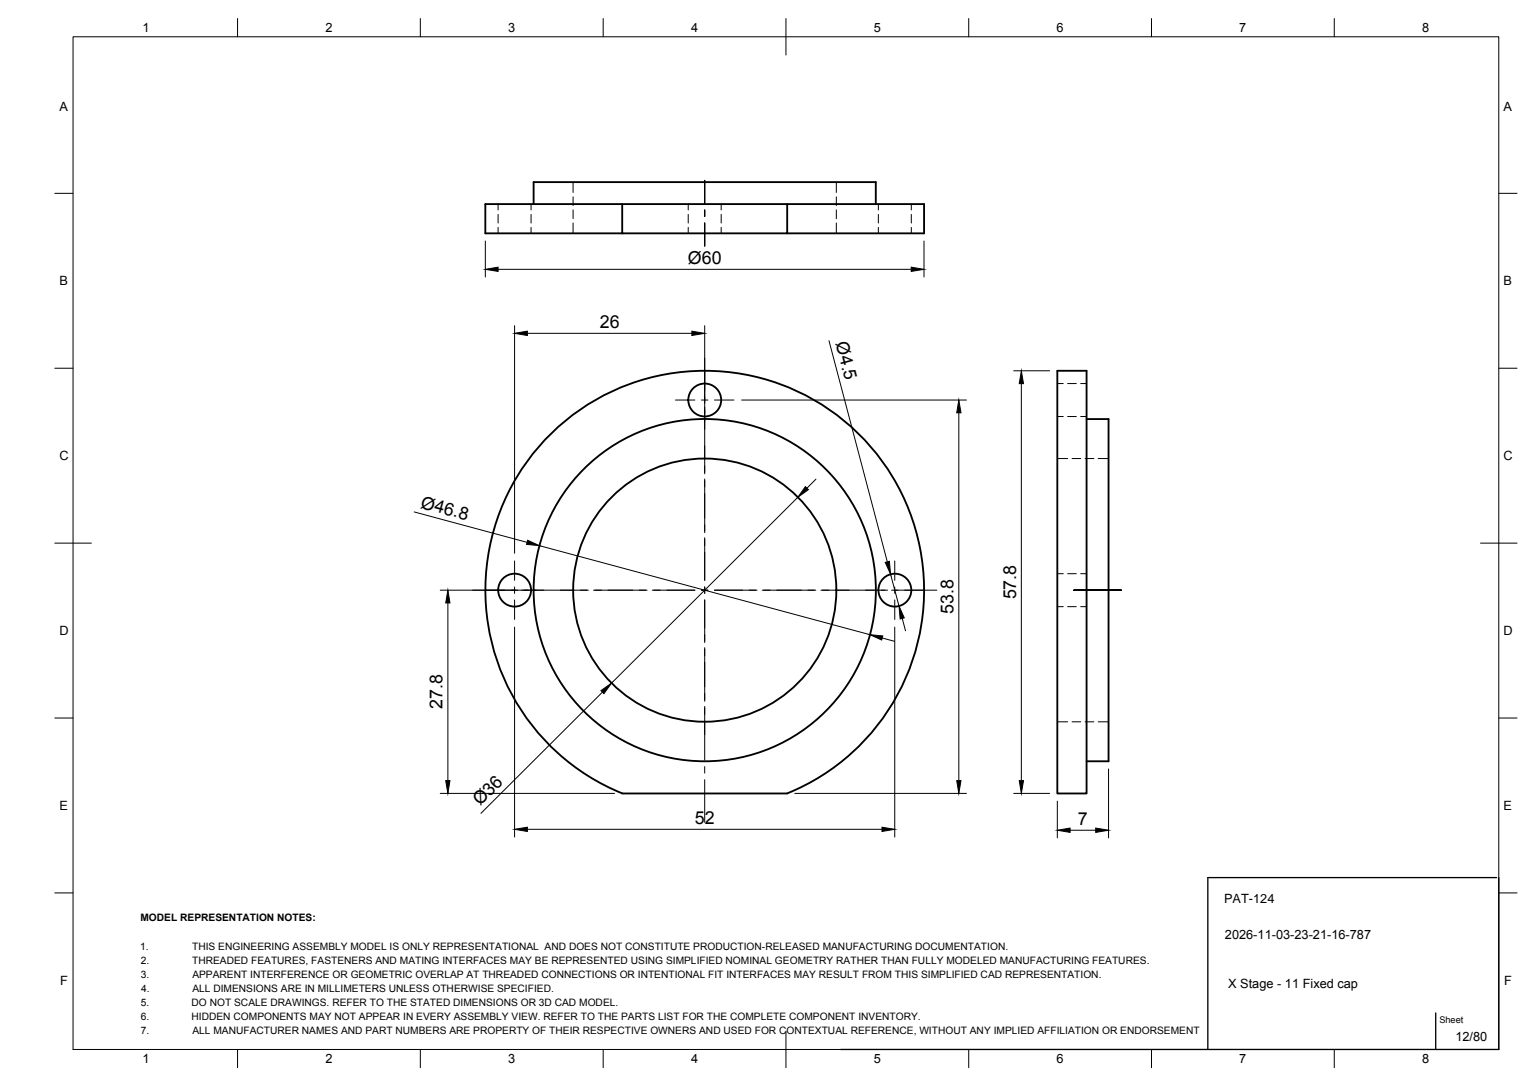
ISO-10303-21;
HEADER;
/* Generated by software containing ST-Developer
 * from STEP Tools, Inc. (www.steptools.com) 
 */

FILE_DESCRIPTION(
/* description */ ('XY cross-slide table'),
/* implementation_level */ '2;1');

FILE_NAME(
/* name */ 'X Stage - 11 Fixed cap.step',
/* time_stamp */ '2026-10-28T03:22:46-07:00',
/* author */ (''),
/* organization */ (''),
/* preprocessor_version */ 'ST-DEVELOPER v20.2',
/* originating_system */ 'Autodesk Translation Framework v15.17.0.0',
/* authorisation */ '');

FILE_SCHEMA (('AUTOMOTIVE_DESIGN { 1 0 10303 214 3 1 1 }'));
ENDSEC;

DATA;
#10=MECHANICAL_DESIGN_GEOMETRIC_PRESENTATION_REPRESENTATION('',(#1677),#62984);
#1511=SHAPE_REPRESENTATION_RELATIONSHIP('SRR','None',#63359,#1594);
#1594=ADVANCED_BREP_SHAPE_REPRESENTATION('',(#1790),#62896);
#1677=STYLED_ITEM('',(#63926),#1790);
#1790=MANIFOLD_SOLID_BREP('Body1',#22971);
#1956=FACE_BOUND('',#4350,.T.);
#1957=FACE_BOUND('',#4351,.T.);
#1958=FACE_BOUND('',#4352,.T.);
#1959=FACE_BOUND('',#4353,.T.);
#1960=FACE_BOUND('',#4357,.T.);
#1961=FACE_BOUND('',#4360,.T.);
#1962=FACE_BOUND('',#4361,.T.);
#1963=FACE_BOUND('',#4362,.T.);
#1964=FACE_BOUND('',#4363,.T.);
#2345=PLANE('',#24201);
#2346=PLANE('',#24202);
#2347=PLANE('',#24209);
#2348=PLANE('',#24213);
#2962=FACE_OUTER_BOUND('',#4345,.T.);
#2963=FACE_OUTER_BOUND('',#4346,.T.);
#2964=FACE_OUTER_BOUND('',#4347,.T.);
#2965=FACE_OUTER_BOUND('',#4348,.T.);
#2966=FACE_OUTER_BOUND('',#4349,.T.);
#2967=FACE_OUTER_BOUND('',#4354,.T.);
#2968=FACE_OUTER_BOUND('',#4355,.T.);
#2969=FACE_OUTER_BOUND('',#4356,.T.);
#2970=FACE_OUTER_BOUND('',#4358,.T.);
#2971=FACE_OUTER_BOUND('',#4359,.T.);
#4345=EDGE_LOOP('',(#15320,#15321,#15322,#15323));
#4346=EDGE_LOOP('',(#15324,#15325,#15326,#15327));
#4347=EDGE_LOOP('',(#15328,#15329,#15330,#15331));
#4348=EDGE_LOOP('',(#15332,#15333,#15334,#15335));
#4349=EDGE_LOOP('',(#15336,#15337));
#4350=EDGE_LOOP('',(#15338));
#4351=EDGE_LOOP('',(#15339));
#4352=EDGE_LOOP('',(#15340));
#4353=EDGE_LOOP('',(#15341));
#4354=EDGE_LOOP('',(#15342,#15343,#15344,#15345));
#4355=EDGE_LOOP('',(#15346,#15347,#15348,#15349));
#4356=EDGE_LOOP('',(#15350));
#4357=EDGE_LOOP('',(#15351));
#4358=EDGE_LOOP('',(#15352,#15353,#15354,#15355));
#4359=EDGE_LOOP('',(#15356,#15357));
#4360=EDGE_LOOP('',(#15358));
#4361=EDGE_LOOP('',(#15359));
#4362=EDGE_LOOP('',(#15360));
#4363=EDGE_LOOP('',(#15361));
#6026=LINE('',#33322,#7513);
#6027=LINE('',#33328,#7514);
#6028=LINE('',#33334,#7515);
#6029=LINE('',#33339,#7516);
#6030=LINE('',#33341,#7517);
#6031=LINE('',#33343,#7518);
#6032=LINE('',#33344,#7519);
#6033=LINE('',#33353,#7520);
#6034=LINE('',#33361,#7521);
#7513=VECTOR('',#26969,0.225);
#7514=VECTOR('',#26976,0.225);
#7515=VECTOR('',#26983,0.225);
#7516=VECTOR('',#26988,1.);
#7517=VECTOR('',#26989,1.);
#7518=VECTOR('',#26990,1.);
#7519=VECTOR('',#26991,1.);
#7520=VECTOR('',#27004,2.34);
#7521=VECTOR('',#27015,1.8);
#8968=CIRCLE('',#24193,0.225);
#8969=CIRCLE('',#24194,0.225);
#8970=CIRCLE('',#24196,0.225);
#8971=CIRCLE('',#24197,0.225);
#8972=CIRCLE('',#24199,0.225);
#8973=CIRCLE('',#24200,0.225);
#8974=CIRCLE('',#24203,3.);
#8975=CIRCLE('',#24204,2.34);
#8976=CIRCLE('',#24206,3.);
#8977=CIRCLE('',#24208,2.34);
#8978=CIRCLE('',#24210,1.8);
#8979=CIRCLE('',#24212,1.8);
#9909=VERTEX_POINT('',#33319);
#9910=VERTEX_POINT('',#33321);
#9911=VERTEX_POINT('',#33325);
#9912=VERTEX_POINT('',#33327);
#9913=VERTEX_POINT('',#33331);
#9914=VERTEX_POINT('',#33333);
#9915=VERTEX_POINT('',#33337);
#9916=VERTEX_POINT('',#33338);
#9917=VERTEX_POINT('',#33340);
#9918=VERTEX_POINT('',#33342);
#9919=VERTEX_POINT('',#33347);
#9920=VERTEX_POINT('',#33352);
#9921=VERTEX_POINT('',#33356);
#9922=VERTEX_POINT('',#33359);
#12044=EDGE_CURVE('',#9909,#9909,#8968,.T.);
#12045=EDGE_CURVE('',#9909,#9910,#6026,.T.);
#12046=EDGE_CURVE('',#9910,#9910,#8969,.T.);
#12047=EDGE_CURVE('',#9911,#9911,#8970,.T.);
#12048=EDGE_CURVE('',#9911,#9912,#6027,.T.);
#12049=EDGE_CURVE('',#9912,#9912,#8971,.T.);
#12050=EDGE_CURVE('',#9913,#9913,#8972,.T.);
#12051=EDGE_CURVE('',#9913,#9914,#6028,.T.);
#12052=EDGE_CURVE('',#9914,#9914,#8973,.T.);
#12053=EDGE_CURVE('',#9915,#9916,#6029,.T.);
#12054=EDGE_CURVE('',#9917,#9915,#6030,.T.);
#12055=EDGE_CURVE('',#9918,#9917,#6031,.T.);
#12056=EDGE_CURVE('',#9916,#9918,#6032,.T.);
#12057=EDGE_CURVE('',#9917,#9915,#8974,.T.);
#12058=EDGE_CURVE('',#9919,#9919,#8975,.T.);
#12059=EDGE_CURVE('',#9918,#9916,#8976,.T.);
#12060=EDGE_CURVE('',#9919,#9920,#6033,.T.);
#12061=EDGE_CURVE('',#9920,#9920,#8977,.T.);
#12062=EDGE_CURVE('',#9921,#9921,#8978,.T.);
#12063=EDGE_CURVE('',#9922,#9922,#8979,.T.);
#12064=EDGE_CURVE('',#9922,#9921,#6034,.T.);
#15320=ORIENTED_EDGE('',*,*,#12044,.F.);
#15321=ORIENTED_EDGE('',*,*,#12045,.T.);
#15322=ORIENTED_EDGE('',*,*,#12046,.F.);
#15323=ORIENTED_EDGE('',*,*,#12045,.F.);
#15324=ORIENTED_EDGE('',*,*,#12047,.F.);
#15325=ORIENTED_EDGE('',*,*,#12048,.T.);
#15326=ORIENTED_EDGE('',*,*,#12049,.F.);
#15327=ORIENTED_EDGE('',*,*,#12048,.F.);
#15328=ORIENTED_EDGE('',*,*,#12050,.F.);
#15329=ORIENTED_EDGE('',*,*,#12051,.T.);
#15330=ORIENTED_EDGE('',*,*,#12052,.F.);
#15331=ORIENTED_EDGE('',*,*,#12051,.F.);
#15332=ORIENTED_EDGE('',*,*,#12053,.F.);
#15333=ORIENTED_EDGE('',*,*,#12054,.F.);
#15334=ORIENTED_EDGE('',*,*,#12055,.F.);
#15335=ORIENTED_EDGE('',*,*,#12056,.F.);
#15336=ORIENTED_EDGE('',*,*,#12054,.T.);
#15337=ORIENTED_EDGE('',*,*,#12057,.F.);
#15338=ORIENTED_EDGE('',*,*,#12044,.T.);
#15339=ORIENTED_EDGE('',*,*,#12047,.T.);
#15340=ORIENTED_EDGE('',*,*,#12050,.T.);
#15341=ORIENTED_EDGE('',*,*,#12058,.T.);
#15342=ORIENTED_EDGE('',*,*,#12055,.T.);
#15343=ORIENTED_EDGE('',*,*,#12057,.T.);
#15344=ORIENTED_EDGE('',*,*,#12053,.T.);
#15345=ORIENTED_EDGE('',*,*,#12059,.F.);
#15346=ORIENTED_EDGE('',*,*,#12058,.F.);
#15347=ORIENTED_EDGE('',*,*,#12060,.T.);
#15348=ORIENTED_EDGE('',*,*,#12061,.T.);
#15349=ORIENTED_EDGE('',*,*,#12060,.F.);
#15350=ORIENTED_EDGE('',*,*,#12061,.F.);
#15351=ORIENTED_EDGE('',*,*,#12062,.F.);
#15352=ORIENTED_EDGE('',*,*,#12063,.F.);
#15353=ORIENTED_EDGE('',*,*,#12064,.T.);
#15354=ORIENTED_EDGE('',*,*,#12062,.T.);
#15355=ORIENTED_EDGE('',*,*,#12064,.F.);
#15356=ORIENTED_EDGE('',*,*,#12056,.T.);
#15357=ORIENTED_EDGE('',*,*,#12059,.T.);
#15358=ORIENTED_EDGE('',*,*,#12046,.T.);
#15359=ORIENTED_EDGE('',*,*,#12049,.T.);
#15360=ORIENTED_EDGE('',*,*,#12052,.T.);
#15361=ORIENTED_EDGE('',*,*,#12063,.T.);
#21084=CYLINDRICAL_SURFACE('',#24192,0.225);
#21085=CYLINDRICAL_SURFACE('',#24195,0.225);
#21086=CYLINDRICAL_SURFACE('',#24198,0.225);
#21087=CYLINDRICAL_SURFACE('',#24205,3.);
#21088=CYLINDRICAL_SURFACE('',#24207,2.34);
#21089=CYLINDRICAL_SURFACE('',#24211,1.8);
#21743=ADVANCED_FACE('',(#2962),#21084,.F.);
#21744=ADVANCED_FACE('',(#2963),#21085,.F.);
#21745=ADVANCED_FACE('',(#2964),#21086,.F.);
#21746=ADVANCED_FACE('',(#2965),#2345,.F.);
#21747=ADVANCED_FACE('',(#2966,#1956,#1957,#1958,#1959),#2346,.F.);
#21748=ADVANCED_FACE('',(#2967),#21087,.T.);
#21749=ADVANCED_FACE('',(#2968),#21088,.T.);
#21750=ADVANCED_FACE('',(#2969,#1960),#2347,.F.);
#21751=ADVANCED_FACE('',(#2970),#21089,.F.);
#21752=ADVANCED_FACE('',(#2971,#1961,#1962,#1963,#1964),#2348,.T.);
#22971=CLOSED_SHELL('',(#21743,#21744,#21745,#21746,#21747,#21748,#21749,
#21750,#21751,#21752));
#24191=AXIS2_PLACEMENT_3D('',#33317,#26963,#26964);
#24192=AXIS2_PLACEMENT_3D('',#33318,#26965,#26966);
#24193=AXIS2_PLACEMENT_3D('',#33320,#26967,#26968);
#24194=AXIS2_PLACEMENT_3D('',#33323,#26970,#26971);
#24195=AXIS2_PLACEMENT_3D('',#33324,#26972,#26973);
#24196=AXIS2_PLACEMENT_3D('',#33326,#26974,#26975);
#24197=AXIS2_PLACEMENT_3D('',#33329,#26977,#26978);
#24198=AXIS2_PLACEMENT_3D('',#33330,#26979,#26980);
#24199=AXIS2_PLACEMENT_3D('',#33332,#26981,#26982);
#24200=AXIS2_PLACEMENT_3D('',#33335,#26984,#26985);
#24201=AXIS2_PLACEMENT_3D('',#33336,#26986,#26987);
#24202=AXIS2_PLACEMENT_3D('',#33345,#26992,#26993);
#24203=AXIS2_PLACEMENT_3D('',#33346,#26994,#26995);
#24204=AXIS2_PLACEMENT_3D('',#33348,#26996,#26997);
#24205=AXIS2_PLACEMENT_3D('',#33349,#26998,#26999);
#24206=AXIS2_PLACEMENT_3D('',#33350,#27000,#27001);
#24207=AXIS2_PLACEMENT_3D('',#33351,#27002,#27003);
#24208=AXIS2_PLACEMENT_3D('',#33354,#27005,#27006);
#24209=AXIS2_PLACEMENT_3D('',#33355,#27007,#27008);
#24210=AXIS2_PLACEMENT_3D('',#33357,#27009,#27010);
#24211=AXIS2_PLACEMENT_3D('',#33358,#27011,#27012);
#24212=AXIS2_PLACEMENT_3D('',#33360,#27013,#27014);
#24213=AXIS2_PLACEMENT_3D('',#33362,#27016,#27017);
#26963=DIRECTION('axis',(0.,0.,1.));
#26964=DIRECTION('refdir',(1.,0.,0.));
#26965=DIRECTION('center_axis',(1.,0.,0.));
#26966=DIRECTION('ref_axis',(0.,0.,-1.));
#26967=DIRECTION('center_axis',(1.,0.,0.));
#26968=DIRECTION('ref_axis',(0.,0.,-1.));
#26969=DIRECTION('',(1.,0.,0.));
#26970=DIRECTION('center_axis',(-1.,0.,0.));
#26971=DIRECTION('ref_axis',(0.,0.,-1.));
#26972=DIRECTION('center_axis',(1.,0.,0.));
#26973=DIRECTION('ref_axis',(0.,0.,-1.));
#26974=DIRECTION('center_axis',(1.,0.,0.));
#26975=DIRECTION('ref_axis',(0.,0.,-1.));
#26976=DIRECTION('',(1.,0.,0.));
#26977=DIRECTION('center_axis',(-1.,0.,0.));
#26978=DIRECTION('ref_axis',(0.,0.,-1.));
#26979=DIRECTION('center_axis',(1.,0.,0.));
#26980=DIRECTION('ref_axis',(0.,0.,-1.));
#26981=DIRECTION('center_axis',(1.,0.,0.));
#26982=DIRECTION('ref_axis',(0.,0.,-1.));
#26983=DIRECTION('',(1.,0.,0.));
#26984=DIRECTION('center_axis',(-1.,0.,0.));
#26985=DIRECTION('ref_axis',(0.,0.,-1.));
#26986=DIRECTION('center_axis',(0.,0.,1.));
#26987=DIRECTION('ref_axis',(0.,-1.,0.));
#26988=DIRECTION('',(1.,0.,0.));
#26989=DIRECTION('',(0.,-1.,0.));
#26990=DIRECTION('',(-1.,0.,0.));
#26991=DIRECTION('',(0.,1.,0.));
#26992=DIRECTION('center_axis',(1.,0.,0.));
#26993=DIRECTION('ref_axis',(0.,0.,-1.));
#26994=DIRECTION('center_axis',(1.,0.,0.));
#26995=DIRECTION('ref_axis',(0.,0.,-1.));
#26996=DIRECTION('center_axis',(1.,0.,0.));
#26997=DIRECTION('ref_axis',(0.,0.,-1.));
#26998=DIRECTION('center_axis',(1.,0.,0.));
#26999=DIRECTION('ref_axis',(0.,1.22464679914735E-16,1.));
#27000=DIRECTION('center_axis',(1.,0.,0.));
#27001=DIRECTION('ref_axis',(0.,0.,-1.));
#27002=DIRECTION('center_axis',(1.,0.,0.));
#27003=DIRECTION('ref_axis',(0.,0.,-1.));
#27004=DIRECTION('',(-1.,0.,0.));
#27005=DIRECTION('center_axis',(1.,0.,0.));
#27006=DIRECTION('ref_axis',(0.,0.,-1.));
#27007=DIRECTION('center_axis',(1.,0.,0.));
#27008=DIRECTION('ref_axis',(0.,0.,-1.));
#27009=DIRECTION('center_axis',(-1.,0.,0.));
#27010=DIRECTION('ref_axis',(0.,0.,-1.));
#27011=DIRECTION('center_axis',(1.,0.,0.));
#27012=DIRECTION('ref_axis',(0.,0.,-1.));
#27013=DIRECTION('center_axis',(-1.,0.,0.));
#27014=DIRECTION('ref_axis',(0.,0.,-1.));
#27015=DIRECTION('',(-1.,0.,0.));
#27016=DIRECTION('center_axis',(1.,0.,0.));
#27017=DIRECTION('ref_axis',(0.,0.,-1.));
#33317=CARTESIAN_POINT('',(0.,0.,0.));
#33318=CARTESIAN_POINT('Origin',(24.9,-2.6,4.));
#33319=CARTESIAN_POINT('',(25.,-2.6,4.225));
#33320=CARTESIAN_POINT('Origin',(25.,-2.6,4.));
#33321=CARTESIAN_POINT('',(25.4,-2.6,4.225));
#33322=CARTESIAN_POINT('',(24.9,-2.6,4.225));
#33323=CARTESIAN_POINT('Origin',(25.4,-2.6,4.));
#33324=CARTESIAN_POINT('Origin',(24.9,2.6,4.));
#33325=CARTESIAN_POINT('',(25.,2.6,4.225));
#33326=CARTESIAN_POINT('Origin',(25.,2.6,4.));
#33327=CARTESIAN_POINT('',(25.4,2.6,4.225));
#33328=CARTESIAN_POINT('',(24.9,2.6,4.225));
#33329=CARTESIAN_POINT('Origin',(25.4,2.6,4.));
#33330=CARTESIAN_POINT('Origin',(24.9,0.,6.6));
#33331=CARTESIAN_POINT('',(25.,-2.75545529808154E-17,6.825));
#33332=CARTESIAN_POINT('Origin',(25.,0.,6.6));
#33333=CARTESIAN_POINT('',(25.4,2.75545529808154E-17,6.825));
#33334=CARTESIAN_POINT('',(24.9,-2.75545529808154E-17,6.825));
#33335=CARTESIAN_POINT('Origin',(25.4,0.,6.6));
#33336=CARTESIAN_POINT('Origin',(24.9,3.5,1.22));
#33337=CARTESIAN_POINT('',(25.,-1.12765242872084,1.22));
#33338=CARTESIAN_POINT('',(25.4,-1.12765242872084,1.22));
#33339=CARTESIAN_POINT('',(25.,-1.12765242872084,1.22));
#33340=CARTESIAN_POINT('',(25.,1.12765242872084,1.22));
#33341=CARTESIAN_POINT('',(25.,1.75,1.22));
#33342=CARTESIAN_POINT('',(25.4,1.12765242872084,1.22));
#33343=CARTESIAN_POINT('',(25.,1.12765242872084,1.22));
#33344=CARTESIAN_POINT('',(25.4,1.75,1.22));
#33345=CARTESIAN_POINT('Origin',(25.,0.,4.));
#33346=CARTESIAN_POINT('Origin',(25.,0.,4.));
#33347=CARTESIAN_POINT('',(25.,-2.86567351000481E-16,6.34));
#33348=CARTESIAN_POINT('Origin',(25.,0.,4.));
#33349=CARTESIAN_POINT('Origin',(25.,0.,4.));
#33350=CARTESIAN_POINT('Origin',(25.4,0.,4.));
#33351=CARTESIAN_POINT('Origin',(24.7,0.,4.));
#33352=CARTESIAN_POINT('',(24.7,-2.86567351000481E-16,6.34));
#33353=CARTESIAN_POINT('',(24.7,-2.86567351000481E-16,6.34));
#33354=CARTESIAN_POINT('Origin',(24.7,0.,4.));
#33355=CARTESIAN_POINT('Origin',(24.7,0.,4.));
#33356=CARTESIAN_POINT('',(24.7,-2.20436423846524E-16,5.8));
#33357=CARTESIAN_POINT('Origin',(24.7,0.,4.));
#33358=CARTESIAN_POINT('Origin',(25.,0.,4.));
#33359=CARTESIAN_POINT('',(25.4,-2.20436423846524E-16,5.8));
#33360=CARTESIAN_POINT('Origin',(25.4,0.,4.));
#33361=CARTESIAN_POINT('',(25.,-2.20436423846524E-16,5.8));
#33362=CARTESIAN_POINT('Origin',(25.4,0.,4.));
#62797=UNCERTAINTY_MEASURE_WITH_UNIT(LENGTH_MEASURE(0.001),#62985,
'DISTANCE_ACCURACY_VALUE',
'Maximum model space distance between geometric entities at asserted c
onnectivities');
#62885=UNCERTAINTY_MEASURE_WITH_UNIT(LENGTH_MEASURE(0.001),#62985,
'DISTANCE_ACCURACY_VALUE',
'Maximum model space distance between geometric entities at asserted c
onnectivities');
#62896=(
GEOMETRIC_REPRESENTATION_CONTEXT(3)
GLOBAL_UNCERTAINTY_ASSIGNED_CONTEXT((#62797))
GLOBAL_UNIT_ASSIGNED_CONTEXT((#62985,#62987,#62988))
REPRESENTATION_CONTEXT('','3D')
);
#62984=(
GEOMETRIC_REPRESENTATION_CONTEXT(3)
GLOBAL_UNCERTAINTY_ASSIGNED_CONTEXT((#62885))
GLOBAL_UNIT_ASSIGNED_CONTEXT((#62985,#62987,#62988))
REPRESENTATION_CONTEXT('','3D')
);
#62985=(
LENGTH_UNIT()
NAMED_UNIT(*)
SI_UNIT(.CENTI.,.METRE.)
);
#62987=(
NAMED_UNIT(*)
PLANE_ANGLE_UNIT()
SI_UNIT($,.RADIAN.)
);
#62988=(
NAMED_UNIT(*)
SI_UNIT($,.STERADIAN.)
SOLID_ANGLE_UNIT()
);
#62999=SHAPE_DEFINITION_REPRESENTATION(#63097,#63359);
#63097=PRODUCT_DEFINITION_SHAPE('',$,#63458);
#63359=SHAPE_REPRESENTATION('',(#24191),#62896);
#63447=PRODUCT_DEFINITION_CONTEXT('part definition',#63743,'design');
#63458=PRODUCT_DEFINITION('X Stage - 11 Fixed cap',
'X Stage - 11 Fixed cap',#63556,#63447);
#63556=PRODUCT_DEFINITION_FORMATION('',$,#63755);
#63743=APPLICATION_CONTEXT(
'Core Data for Automotive Mechanical Design Process');
#63744=PRODUCT_CONTEXT('part definition',#63743,'mechanical');
#63755=PRODUCT('X Stage - 11 Fixed cap','X Stage - 11 Fixed cap',
'X Stage - 11 Fixed cap',(#63744));
#63920=COLOUR_RGB('Off White',0.89,0.88,0.83);
#63921=FILL_AREA_STYLE_COLOUR('',#63920);
#63922=FILL_AREA_STYLE('',(#63921));
#63923=SURFACE_STYLE_FILL_AREA(#63922);
#63924=SURFACE_SIDE_STYLE('',(#63923));
#63925=SURFACE_STYLE_USAGE(.BOTH.,#63924);
#63926=PRESENTATION_STYLE_ASSIGNMENT((#63925));
ENDSEC;
END-ISO-10303-21;
